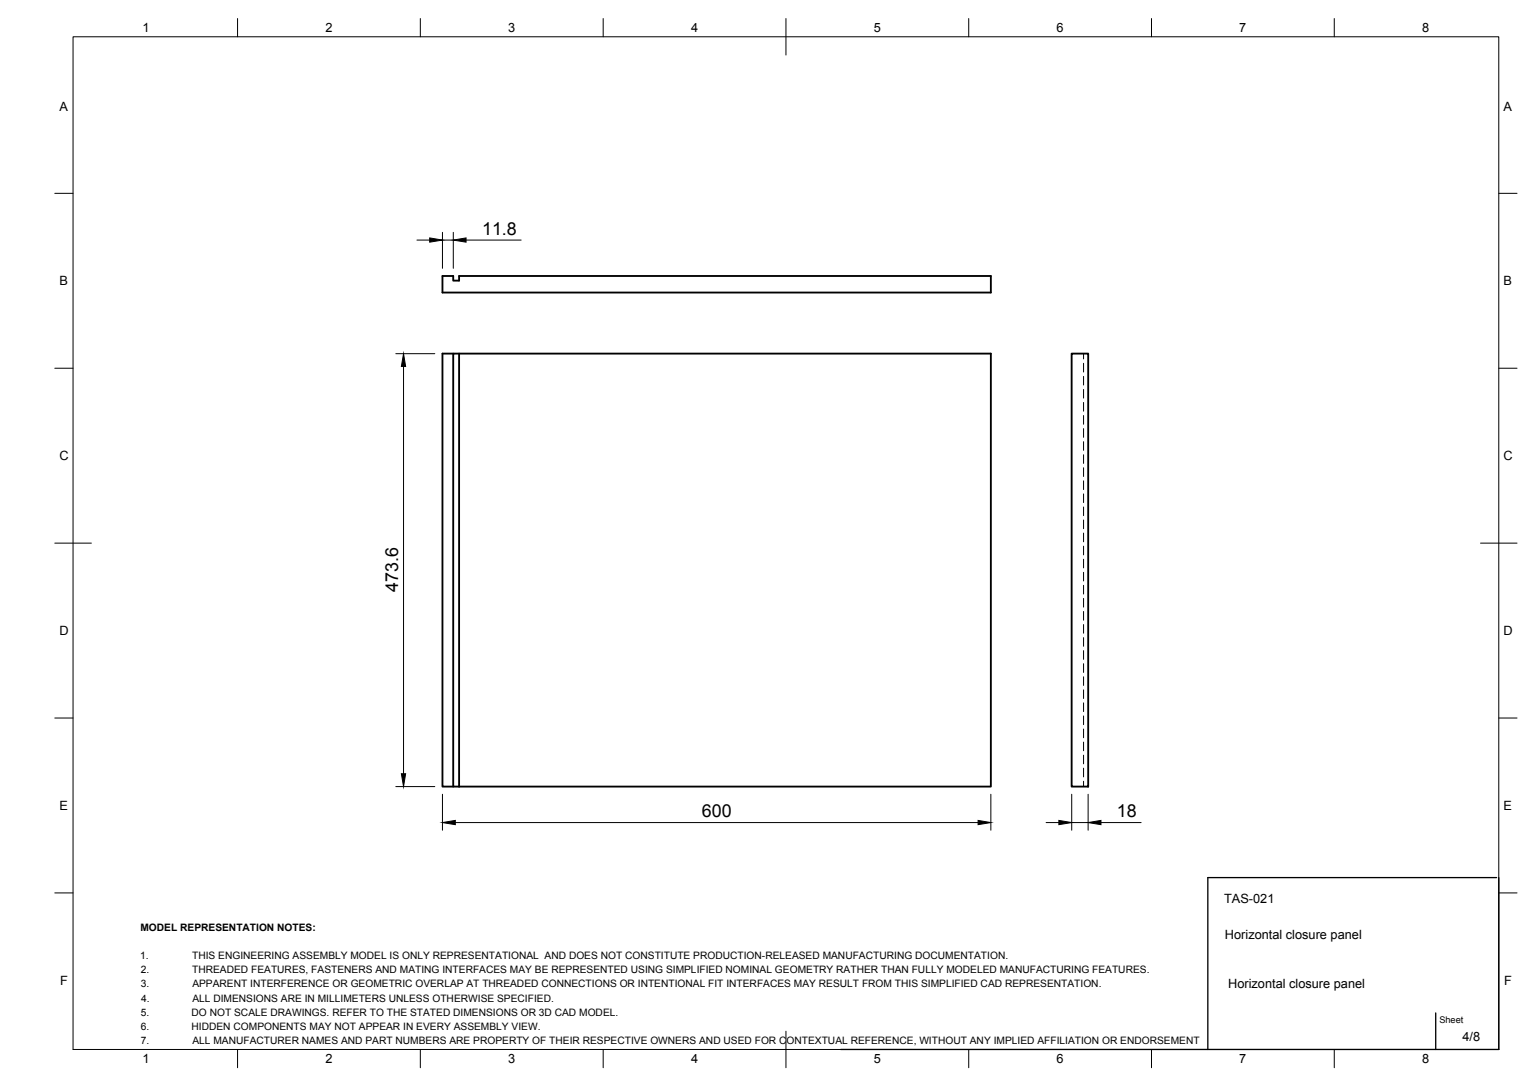
ISO-10303-21;
HEADER;
/* Generated by software containing ST-Developer
 * from STEP Tools, Inc. (www.steptools.com) 
 */

FILE_DESCRIPTION(
/* description */ (''),
/* implementation_level */ '2;1');

FILE_NAME(
/* name */ 'Horizontal closure panel.step',
/* time_stamp */ '2026-11-15T17:48:08-08:00',
/* author */ (''),
/* organization */ (''),
/* preprocessor_version */ 'ST-DEVELOPER v20.2',
/* originating_system */ 'Autodesk Translation Framework v15.17.0.0',
/* authorisation */ '');

FILE_SCHEMA (('AUTOMOTIVE_DESIGN { 1 0 10303 214 3 1 1 }'));
ENDSEC;

DATA;
#10=MECHANICAL_DESIGN_GEOMETRIC_PRESENTATION_REPRESENTATION('',(#140),#2097);
#128=SHAPE_REPRESENTATION_RELATIONSHIP('SRR','None',#2147,#134);
#134=ADVANCED_BREP_SHAPE_REPRESENTATION('',(#146),#2092);
#140=STYLED_ITEM('',(#2186),#146);
#146=MANIFOLD_SOLID_BREP('Body1',#1194);
#187=PLANE('',#1315);
#188=PLANE('',#1316);
#189=PLANE('',#1317);
#190=PLANE('',#1318);
#191=PLANE('',#1319);
#192=PLANE('',#1320);
#193=PLANE('',#1321);
#194=PLANE('',#1322);
#195=PLANE('',#1323);
#196=PLANE('',#1324);
#249=FACE_OUTER_BOUND('',#321,.T.);
#250=FACE_OUTER_BOUND('',#322,.T.);
#251=FACE_OUTER_BOUND('',#323,.T.);
#252=FACE_OUTER_BOUND('',#324,.T.);
#253=FACE_OUTER_BOUND('',#325,.T.);
#254=FACE_OUTER_BOUND('',#326,.T.);
#255=FACE_OUTER_BOUND('',#327,.T.);
#256=FACE_OUTER_BOUND('',#328,.T.);
#257=FACE_OUTER_BOUND('',#329,.T.);
#258=FACE_OUTER_BOUND('',#330,.T.);
#321=EDGE_LOOP('',(#997,#998,#999,#1000));
#322=EDGE_LOOP('',(#1001,#1002,#1003,#1004));
#323=EDGE_LOOP('',(#1005,#1006,#1007,#1008));
#324=EDGE_LOOP('',(#1009,#1010,#1011,#1012,#1013,#1014,#1015,#1016));
#325=EDGE_LOOP('',(#1017,#1018,#1019,#1020));
#326=EDGE_LOOP('',(#1021,#1022,#1023,#1024));
#327=EDGE_LOOP('',(#1025,#1026,#1027,#1028));
#328=EDGE_LOOP('',(#1029,#1030,#1031,#1032,#1033,#1034,#1035,#1036));
#329=EDGE_LOOP('',(#1037,#1038,#1039,#1040));
#330=EDGE_LOOP('',(#1041,#1042,#1043,#1044));
#421=LINE('',#1920,#539);
#422=LINE('',#1922,#540);
#423=LINE('',#1924,#541);
#424=LINE('',#1925,#542);
#425=LINE('',#1929,#543);
#426=LINE('',#1931,#544);
#427=LINE('',#1933,#545);
#428=LINE('',#1934,#546);
#429=LINE('',#1936,#547);
#430=LINE('',#1937,#548);
#431=LINE('',#1940,#549);
#432=LINE('',#1942,#550);
#433=LINE('',#1944,#551);
#434=LINE('',#1946,#552);
#435=LINE('',#1947,#553);
#436=LINE('',#1950,#554);
#437=LINE('',#1951,#555);
#438=LINE('',#1954,#556);
#439=LINE('',#1956,#557);
#440=LINE('',#1957,#558);
#441=LINE('',#1960,#559);
#442=LINE('',#1961,#560);
#443=LINE('',#1963,#561);
#444=LINE('',#1964,#562);
#539=VECTOR('',#1554,1.);
#540=VECTOR('',#1555,1.);
#541=VECTOR('',#1556,1.);
#542=VECTOR('',#1557,1.);
#543=VECTOR('',#1560,1.);
#544=VECTOR('',#1561,1.);
#545=VECTOR('',#1562,1.);
#546=VECTOR('',#1563,1.);
#547=VECTOR('',#1566,1.);
#548=VECTOR('',#1567,1.);
#549=VECTOR('',#1570,1.);
#550=VECTOR('',#1571,1.);
#551=VECTOR('',#1572,1.);
#552=VECTOR('',#1573,1.);
#553=VECTOR('',#1574,1.);
#554=VECTOR('',#1577,1.);
#555=VECTOR('',#1578,1.);
#556=VECTOR('',#1581,1.);
#557=VECTOR('',#1582,1.);
#558=VECTOR('',#1583,1.);
#559=VECTOR('',#1586,1.);
#560=VECTOR('',#1587,1.);
#561=VECTOR('',#1590,1.);
#562=VECTOR('',#1591,1.);
#663=VERTEX_POINT('',#1918);
#664=VERTEX_POINT('',#1919);
#665=VERTEX_POINT('',#1921);
#666=VERTEX_POINT('',#1923);
#667=VERTEX_POINT('',#1927);
#668=VERTEX_POINT('',#1928);
#669=VERTEX_POINT('',#1930);
#670=VERTEX_POINT('',#1932);
#671=VERTEX_POINT('',#1939);
#672=VERTEX_POINT('',#1941);
#673=VERTEX_POINT('',#1943);
#674=VERTEX_POINT('',#1945);
#675=VERTEX_POINT('',#1949);
#676=VERTEX_POINT('',#1953);
#677=VERTEX_POINT('',#1955);
#678=VERTEX_POINT('',#1959);
#781=EDGE_CURVE('',#663,#664,#421,.T.);
#782=EDGE_CURVE('',#665,#663,#422,.T.);
#783=EDGE_CURVE('',#666,#665,#423,.T.);
#784=EDGE_CURVE('',#664,#666,#424,.T.);
#785=EDGE_CURVE('',#667,#668,#425,.T.);
#786=EDGE_CURVE('',#669,#667,#426,.T.);
#787=EDGE_CURVE('',#670,#669,#427,.T.);
#788=EDGE_CURVE('',#668,#670,#428,.T.);
#789=EDGE_CURVE('',#666,#669,#429,.T.);
#790=EDGE_CURVE('',#670,#665,#430,.T.);
#791=EDGE_CURVE('',#671,#663,#431,.T.);
#792=EDGE_CURVE('',#672,#671,#432,.T.);
#793=EDGE_CURVE('',#672,#673,#433,.T.);
#794=EDGE_CURVE('',#673,#674,#434,.T.);
#795=EDGE_CURVE('',#668,#674,#435,.T.);
#796=EDGE_CURVE('',#664,#675,#436,.T.);
#797=EDGE_CURVE('',#675,#671,#437,.T.);
#798=EDGE_CURVE('',#673,#676,#438,.T.);
#799=EDGE_CURVE('',#676,#677,#439,.T.);
#800=EDGE_CURVE('',#674,#677,#440,.T.);
#801=EDGE_CURVE('',#678,#672,#441,.T.);
#802=EDGE_CURVE('',#678,#675,#442,.T.);
#803=EDGE_CURVE('',#677,#667,#443,.T.);
#804=EDGE_CURVE('',#676,#678,#444,.T.);
#997=ORIENTED_EDGE('',*,*,#781,.F.);
#998=ORIENTED_EDGE('',*,*,#782,.F.);
#999=ORIENTED_EDGE('',*,*,#783,.F.);
#1000=ORIENTED_EDGE('',*,*,#784,.F.);
#1001=ORIENTED_EDGE('',*,*,#785,.F.);
#1002=ORIENTED_EDGE('',*,*,#786,.F.);
#1003=ORIENTED_EDGE('',*,*,#787,.F.);
#1004=ORIENTED_EDGE('',*,*,#788,.F.);
#1005=ORIENTED_EDGE('',*,*,#789,.F.);
#1006=ORIENTED_EDGE('',*,*,#783,.T.);
#1007=ORIENTED_EDGE('',*,*,#790,.F.);
#1008=ORIENTED_EDGE('',*,*,#787,.T.);
#1009=ORIENTED_EDGE('',*,*,#788,.T.);
#1010=ORIENTED_EDGE('',*,*,#790,.T.);
#1011=ORIENTED_EDGE('',*,*,#782,.T.);
#1012=ORIENTED_EDGE('',*,*,#791,.F.);
#1013=ORIENTED_EDGE('',*,*,#792,.F.);
#1014=ORIENTED_EDGE('',*,*,#793,.T.);
#1015=ORIENTED_EDGE('',*,*,#794,.T.);
#1016=ORIENTED_EDGE('',*,*,#795,.F.);
#1017=ORIENTED_EDGE('',*,*,#781,.T.);
#1018=ORIENTED_EDGE('',*,*,#796,.T.);
#1019=ORIENTED_EDGE('',*,*,#797,.T.);
#1020=ORIENTED_EDGE('',*,*,#791,.T.);
#1021=ORIENTED_EDGE('',*,*,#798,.T.);
#1022=ORIENTED_EDGE('',*,*,#799,.T.);
#1023=ORIENTED_EDGE('',*,*,#800,.F.);
#1024=ORIENTED_EDGE('',*,*,#794,.F.);
#1025=ORIENTED_EDGE('',*,*,#801,.T.);
#1026=ORIENTED_EDGE('',*,*,#792,.T.);
#1027=ORIENTED_EDGE('',*,*,#797,.F.);
#1028=ORIENTED_EDGE('',*,*,#802,.F.);
#1029=ORIENTED_EDGE('',*,*,#786,.T.);
#1030=ORIENTED_EDGE('',*,*,#803,.F.);
#1031=ORIENTED_EDGE('',*,*,#799,.F.);
#1032=ORIENTED_EDGE('',*,*,#804,.T.);
#1033=ORIENTED_EDGE('',*,*,#802,.T.);
#1034=ORIENTED_EDGE('',*,*,#796,.F.);
#1035=ORIENTED_EDGE('',*,*,#784,.T.);
#1036=ORIENTED_EDGE('',*,*,#789,.T.);
#1037=ORIENTED_EDGE('',*,*,#785,.T.);
#1038=ORIENTED_EDGE('',*,*,#795,.T.);
#1039=ORIENTED_EDGE('',*,*,#800,.T.);
#1040=ORIENTED_EDGE('',*,*,#803,.T.);
#1041=ORIENTED_EDGE('',*,*,#804,.F.);
#1042=ORIENTED_EDGE('',*,*,#798,.F.);
#1043=ORIENTED_EDGE('',*,*,#793,.F.);
#1044=ORIENTED_EDGE('',*,*,#801,.F.);
#1161=ADVANCED_FACE('',(#249),#187,.F.);
#1162=ADVANCED_FACE('',(#250),#188,.F.);
#1163=ADVANCED_FACE('',(#251),#189,.T.);
#1164=ADVANCED_FACE('',(#252),#190,.T.);
#1165=ADVANCED_FACE('',(#253),#191,.T.);
#1166=ADVANCED_FACE('',(#254),#192,.T.);
#1167=ADVANCED_FACE('',(#255),#193,.T.);
#1168=ADVANCED_FACE('',(#256),#194,.T.);
#1169=ADVANCED_FACE('',(#257),#195,.T.);
#1170=ADVANCED_FACE('',(#258),#196,.F.);
#1194=CLOSED_SHELL('',(#1161,#1162,#1163,#1164,#1165,#1166,#1167,#1168,
#1169,#1170));
#1314=AXIS2_PLACEMENT_3D('',#1916,#1550,#1551);
#1315=AXIS2_PLACEMENT_3D('',#1917,#1552,#1553);
#1316=AXIS2_PLACEMENT_3D('',#1926,#1558,#1559);
#1317=AXIS2_PLACEMENT_3D('',#1935,#1564,#1565);
#1318=AXIS2_PLACEMENT_3D('',#1938,#1568,#1569);
#1319=AXIS2_PLACEMENT_3D('',#1948,#1575,#1576);
#1320=AXIS2_PLACEMENT_3D('',#1952,#1579,#1580);
#1321=AXIS2_PLACEMENT_3D('',#1958,#1584,#1585);
#1322=AXIS2_PLACEMENT_3D('',#1962,#1588,#1589);
#1323=AXIS2_PLACEMENT_3D('',#1965,#1592,#1593);
#1324=AXIS2_PLACEMENT_3D('',#1966,#1594,#1595);
#1550=DIRECTION('axis',(0.,0.,1.));
#1551=DIRECTION('refdir',(1.,0.,0.));
#1552=DIRECTION('center_axis',(0.,-1.,0.));
#1553=DIRECTION('ref_axis',(1.,0.,0.));
#1554=DIRECTION('',(-1.,0.,0.));
#1555=DIRECTION('',(0.,0.,1.));
#1556=DIRECTION('',(1.,0.,0.));
#1557=DIRECTION('',(0.,0.,-1.));
#1558=DIRECTION('center_axis',(0.,1.,0.));
#1559=DIRECTION('ref_axis',(-1.,0.,0.));
#1560=DIRECTION('',(1.,0.,0.));
#1561=DIRECTION('',(0.,0.,1.));
#1562=DIRECTION('',(-1.,0.,0.));
#1563=DIRECTION('',(0.,0.,-1.));
#1564=DIRECTION('center_axis',(0.,0.,1.));
#1565=DIRECTION('ref_axis',(1.,0.,0.));
#1566=DIRECTION('',(0.,1.,0.));
#1567=DIRECTION('',(0.,-1.,0.));
#1568=DIRECTION('center_axis',(1.,0.,0.));
#1569=DIRECTION('ref_axis',(0.,1.,0.));
#1570=DIRECTION('',(0.,1.,0.));
#1571=DIRECTION('',(0.,0.,1.));
#1572=DIRECTION('',(0.,1.,0.));
#1573=DIRECTION('',(0.,0.,1.));
#1574=DIRECTION('',(0.,1.,0.));
#1575=DIRECTION('center_axis',(0.,0.,1.));
#1576=DIRECTION('ref_axis',(1.,0.,0.));
#1577=DIRECTION('',(0.,-1.,0.));
#1578=DIRECTION('',(1.,0.,0.));
#1579=DIRECTION('center_axis',(0.,1.,0.));
#1580=DIRECTION('ref_axis',(-1.,0.,0.));
#1581=DIRECTION('',(-1.,0.,0.));
#1582=DIRECTION('',(0.,0.,1.));
#1583=DIRECTION('',(-1.,0.,0.));
#1584=DIRECTION('center_axis',(0.,-1.,0.));
#1585=DIRECTION('ref_axis',(1.,0.,0.));
#1586=DIRECTION('',(1.,0.,0.));
#1587=DIRECTION('',(0.,0.,1.));
#1588=DIRECTION('center_axis',(-1.,0.,0.));
#1589=DIRECTION('ref_axis',(0.,-1.,0.));
#1590=DIRECTION('',(0.,-1.,0.));
#1591=DIRECTION('',(0.,-1.,0.));
#1592=DIRECTION('center_axis',(0.,0.,1.));
#1593=DIRECTION('ref_axis',(1.,0.,0.));
#1594=DIRECTION('center_axis',(0.,0.,1.));
#1595=DIRECTION('ref_axis',(1.,0.,0.));
#1916=CARTESIAN_POINT('',(0.,0.,0.));
#1917=CARTESIAN_POINT('Origin',(0.,58.18,1.3));
#1918=CARTESIAN_POINT('',(47.36,58.18,1.8));
#1919=CARTESIAN_POINT('',(0.,58.18,1.8));
#1920=CARTESIAN_POINT('',(11.84,58.18,1.8));
#1921=CARTESIAN_POINT('',(47.36,58.18,1.3));
#1922=CARTESIAN_POINT('',(47.36,58.18,0.65));
#1923=CARTESIAN_POINT('',(0.,58.18,1.3));
#1924=CARTESIAN_POINT('',(0.,58.18,1.3));
#1925=CARTESIAN_POINT('',(0.,58.18,0.65));
#1926=CARTESIAN_POINT('Origin',(47.36,58.82,1.3));
#1927=CARTESIAN_POINT('',(0.,58.82,1.8));
#1928=CARTESIAN_POINT('',(47.36,58.82,1.8));
#1929=CARTESIAN_POINT('',(35.52,58.82,1.8));
#1930=CARTESIAN_POINT('',(0.,58.82,1.3));
#1931=CARTESIAN_POINT('',(0.,58.82,0.65));
#1932=CARTESIAN_POINT('',(47.36,58.82,1.3));
#1933=CARTESIAN_POINT('',(47.36,58.82,1.3));
#1934=CARTESIAN_POINT('',(47.36,58.82,0.65));
#1935=CARTESIAN_POINT('Origin',(23.68,58.5,1.3));
#1936=CARTESIAN_POINT('',(0.,59.25,1.3));
#1937=CARTESIAN_POINT('',(47.36,29.25,1.3));
#1938=CARTESIAN_POINT('Origin',(47.36,0.,0.));
#1939=CARTESIAN_POINT('',(47.36,0.,1.8));
#1940=CARTESIAN_POINT('',(47.36,0.,1.8));
#1941=CARTESIAN_POINT('',(47.36,0.,0.));
#1942=CARTESIAN_POINT('',(47.36,0.,0.));
#1943=CARTESIAN_POINT('',(47.36,60.,0.));
#1944=CARTESIAN_POINT('',(47.36,0.,0.));
#1945=CARTESIAN_POINT('',(47.36,60.,1.8));
#1946=CARTESIAN_POINT('',(47.36,60.,0.));
#1947=CARTESIAN_POINT('',(47.36,0.,1.8));
#1948=CARTESIAN_POINT('Origin',(23.68,30.,1.8));
#1949=CARTESIAN_POINT('',(0.,0.,1.8));
#1950=CARTESIAN_POINT('',(0.,60.,1.8));
#1951=CARTESIAN_POINT('',(0.,0.,1.8));
#1952=CARTESIAN_POINT('Origin',(47.36,60.,0.));
#1953=CARTESIAN_POINT('',(0.,60.,0.));
#1954=CARTESIAN_POINT('',(47.36,60.,0.));
#1955=CARTESIAN_POINT('',(0.,60.,1.8));
#1956=CARTESIAN_POINT('',(0.,60.,0.));
#1957=CARTESIAN_POINT('',(47.36,60.,1.8));
#1958=CARTESIAN_POINT('Origin',(0.,0.,0.));
#1959=CARTESIAN_POINT('',(0.,0.,0.));
#1960=CARTESIAN_POINT('',(0.,0.,0.));
#1961=CARTESIAN_POINT('',(0.,0.,0.));
#1962=CARTESIAN_POINT('Origin',(0.,60.,0.));
#1963=CARTESIAN_POINT('',(0.,60.,1.8));
#1964=CARTESIAN_POINT('',(0.,60.,0.));
#1965=CARTESIAN_POINT('Origin',(23.68,30.,1.8));
#1966=CARTESIAN_POINT('Origin',(23.68,30.,0.));
#2084=UNCERTAINTY_MEASURE_WITH_UNIT(LENGTH_MEASURE(0.001),#2098,
'DISTANCE_ACCURACY_VALUE',
'Maximum model space distance between geometric entities at asserted c
onnectivities');
#2089=UNCERTAINTY_MEASURE_WITH_UNIT(LENGTH_MEASURE(0.001),#2098,
'DISTANCE_ACCURACY_VALUE',
'Maximum model space distance between geometric entities at asserted c
onnectivities');
#2092=(
GEOMETRIC_REPRESENTATION_CONTEXT(3)
GLOBAL_UNCERTAINTY_ASSIGNED_CONTEXT((#2084))
GLOBAL_UNIT_ASSIGNED_CONTEXT((#2098,#2100,#2101))
REPRESENTATION_CONTEXT('','3D')
);
#2097=(
GEOMETRIC_REPRESENTATION_CONTEXT(3)
GLOBAL_UNCERTAINTY_ASSIGNED_CONTEXT((#2089))
GLOBAL_UNIT_ASSIGNED_CONTEXT((#2098,#2100,#2101))
REPRESENTATION_CONTEXT('','3D')
);
#2098=(
LENGTH_UNIT()
NAMED_UNIT(*)
SI_UNIT(.CENTI.,.METRE.)
);
#2100=(
NAMED_UNIT(*)
PLANE_ANGLE_UNIT()
SI_UNIT($,.RADIAN.)
);
#2101=(
NAMED_UNIT(*)
SI_UNIT($,.STERADIAN.)
SOLID_ANGLE_UNIT()
);
#2104=SHAPE_DEFINITION_REPRESENTATION(#2111,#2147);
#2111=PRODUCT_DEFINITION_SHAPE('',$,#2155);
#2147=SHAPE_REPRESENTATION('',(#1314),#2092);
#2152=PRODUCT_DEFINITION_CONTEXT('part definition',#2175,'design');
#2155=PRODUCT_DEFINITION('Horizontal closure panel',
'Horizontal closure panel',#2162,#2152);
#2162=PRODUCT_DEFINITION_FORMATION('',$,#2179);
#2175=APPLICATION_CONTEXT(
'Core Data for Automotive Mechanical Design Process');
#2176=PRODUCT_CONTEXT('part definition',#2175,'mechanical');
#2179=PRODUCT('Horizontal closure panel','Horizontal closure panel',$,(#2176));
#2186=PRESENTATION_STYLE_ASSIGNMENT((#2193));
#2193=SURFACE_STYLE_USAGE(.BOTH.,#2200);
#2200=SURFACE_SIDE_STYLE('',(#2207));
#2207=SURFACE_STYLE_FILL_AREA(#2214);
#2214=FILL_AREA_STYLE('Horizontal closure panel finish',(#2221));
#2221=FILL_AREA_STYLE_COLOUR('Horizontal closure panel finish',#2228);
#2228=COLOUR_RGB('Horizontal closure panel finish',0.662745098039216,0.823529411764706,
0.917647058823529);
ENDSEC;
END-ISO-10303-21;
